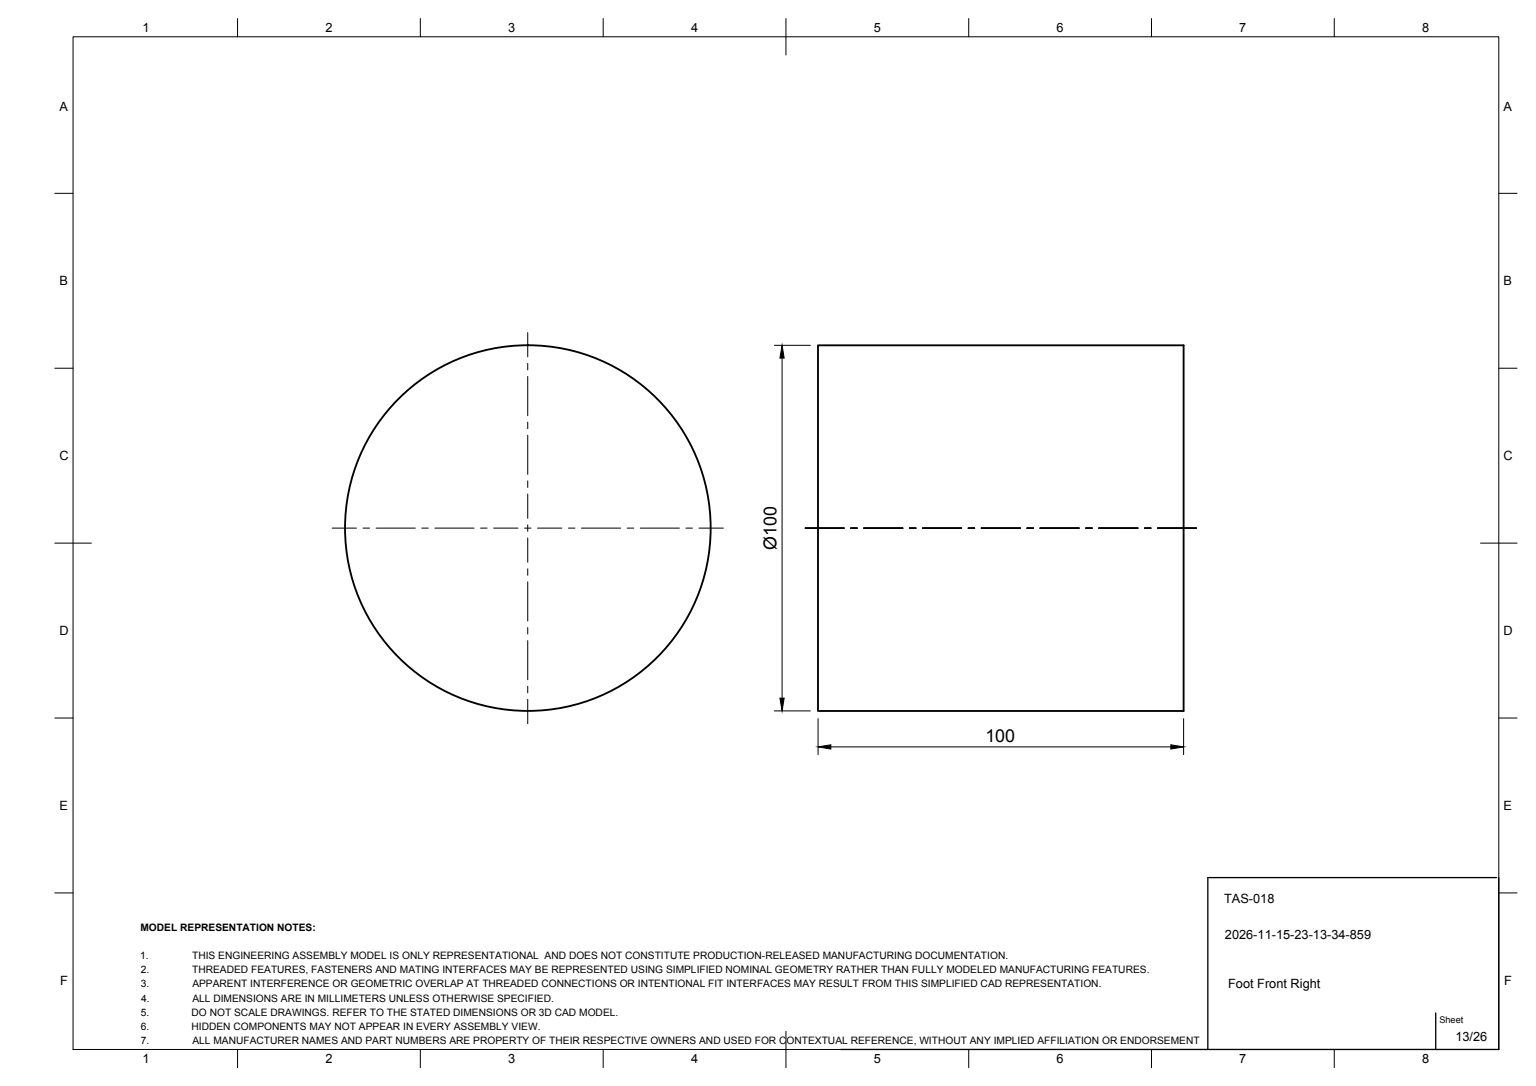
ISO-10303-21;
HEADER;
/* Generated by software containing ST-Developer
 * from STEP Tools, Inc. (www.steptools.com) 
 */

FILE_DESCRIPTION(
/* description */ (''),
/* implementation_level */ '2;1');

FILE_NAME(
/* name */ 'Foot Front Right.step',
/* time_stamp */ '2026-11-15T15:17:57-08:00',
/* author */ (''),
/* organization */ (''),
/* preprocessor_version */ 'ST-DEVELOPER v20.2',
/* originating_system */ 'Autodesk Translation Framework v15.17.0.0',
/* authorisation */ '');

FILE_SCHEMA (('AUTOMOTIVE_DESIGN { 1 0 10303 214 3 1 1 }'));
ENDSEC;

DATA;
#10=MECHANICAL_DESIGN_GEOMETRIC_PRESENTATION_REPRESENTATION('',(#188),#3723);
#13=CIRCLE('',#2395,1.96850393700787);
#14=CIRCLE('',#2396,1.96850393700787);
#24=CYLINDRICAL_SURFACE('',#2394,1.96850393700787);
#140=SHAPE_REPRESENTATION_RELATIONSHIP('SRR','None',#3821,#164);
#164=ADVANCED_BREP_SHAPE_REPRESENTATION('',(#212),#3710);
#188=STYLED_ITEM('',(#3945),#212);
#212=MANIFOLD_SOLID_BREP('Body1',#2036);
#288=FACE_OUTER_BOUND('',#414,.T.);
#289=FACE_OUTER_BOUND('',#415,.T.);
#290=FACE_OUTER_BOUND('',#416,.T.);
#414=EDGE_LOOP('',(#1557,#1558,#1559,#1560));
#415=EDGE_LOOP('',(#1561));
#416=EDGE_LOOP('',(#1562));
#598=LINE('',#3390,#820);
#820=VECTOR('',#2788,1.96850393700787);
#1003=VERTEX_POINT('',#3387);
#1004=VERTEX_POINT('',#3389);
#1200=EDGE_CURVE('',#1003,#1003,#13,.T.);
#1201=EDGE_CURVE('',#1003,#1004,#598,.T.);
#1202=EDGE_CURVE('',#1004,#1004,#14,.T.);
#1557=ORIENTED_EDGE('',*,*,#1200,.T.);
#1558=ORIENTED_EDGE('',*,*,#1201,.T.);
#1559=ORIENTED_EDGE('',*,*,#1202,.F.);
#1560=ORIENTED_EDGE('',*,*,#1201,.F.);
#1561=ORIENTED_EDGE('',*,*,#1202,.T.);
#1562=ORIENTED_EDGE('',*,*,#1200,.F.);
#1841=PLANE('',#2397);
#1842=PLANE('',#2398);
#1962=ADVANCED_FACE('',(#288),#24,.T.);
#1963=ADVANCED_FACE('',(#289),#1841,.T.);
#1964=ADVANCED_FACE('',(#290),#1842,.F.);
#2036=CLOSED_SHELL('',(#1962,#1963,#1964));
#2393=AXIS2_PLACEMENT_3D('',#3385,#2782,#2783);
#2394=AXIS2_PLACEMENT_3D('',#3386,#2784,#2785);
#2395=AXIS2_PLACEMENT_3D('',#3388,#2786,#2787);
#2396=AXIS2_PLACEMENT_3D('',#3391,#2789,#2790);
#2397=AXIS2_PLACEMENT_3D('',#3392,#2791,#2792);
#2398=AXIS2_PLACEMENT_3D('',#3393,#2793,#2794);
#2782=DIRECTION('axis',(0.,0.,1.));
#2783=DIRECTION('refdir',(1.,0.,0.));
#2784=DIRECTION('center_axis',(0.,1.,0.));
#2785=DIRECTION('ref_axis',(0.,0.,1.));
#2786=DIRECTION('center_axis',(0.,-1.,0.));
#2787=DIRECTION('ref_axis',(0.,0.,-1.));
#2788=DIRECTION('',(0.,-1.,0.));
#2789=DIRECTION('center_axis',(0.,-1.,0.));
#2790=DIRECTION('ref_axis',(0.,0.,-1.));
#2791=DIRECTION('center_axis',(0.,-1.,0.));
#2792=DIRECTION('ref_axis',(0.,0.,-1.));
#2793=DIRECTION('center_axis',(0.,-1.,0.));
#2794=DIRECTION('ref_axis',(0.,0.,-1.));
#3385=CARTESIAN_POINT('',(0.,0.,0.));
#3386=CARTESIAN_POINT('Origin',(33.6377952755905,-4.91732638859567E-15,
19.6377952755906));
#3387=CARTESIAN_POINT('',(33.6377952755905,3.93700787401574,17.6692913385827));
#3388=CARTESIAN_POINT('Origin',(33.6377952755905,3.93700787401574,19.6377952755906));
#3389=CARTESIAN_POINT('',(33.6377952755905,-4.91732638859567E-15,17.6692913385827));
#3390=CARTESIAN_POINT('',(33.6377952755905,-4.91732638859567E-15,17.6692913385827));
#3391=CARTESIAN_POINT('Origin',(33.6377952755905,-4.91732638859567E-15,
19.6377952755906));
#3392=CARTESIAN_POINT('Origin',(33.6377952755905,-4.91732638859567E-15,
19.6377952755906));
#3393=CARTESIAN_POINT('Origin',(33.6377952755905,3.93700787401574,19.6377952755906));
#3683=UNCERTAINTY_MEASURE_WITH_UNIT(LENGTH_MEASURE(0.000393700787401575),
#3725,'DISTANCE_ACCURACY_VALUE',
'Maximum model space distance between geometric entities at asserted c
onnectivities');
#3696=UNCERTAINTY_MEASURE_WITH_UNIT(LENGTH_MEASURE(0.000393700787401575),
#3725,'DISTANCE_ACCURACY_VALUE',
'Maximum model space distance between geometric entities at asserted c
onnectivities');
#3710=(
GEOMETRIC_REPRESENTATION_CONTEXT(3)
GLOBAL_UNCERTAINTY_ASSIGNED_CONTEXT((#3683))
GLOBAL_UNIT_ASSIGNED_CONTEXT((#3725,#3729,#3730))
REPRESENTATION_CONTEXT('','3D')
);
#3723=(
GEOMETRIC_REPRESENTATION_CONTEXT(3)
GLOBAL_UNCERTAINTY_ASSIGNED_CONTEXT((#3696))
GLOBAL_UNIT_ASSIGNED_CONTEXT((#3725,#3729,#3730))
REPRESENTATION_CONTEXT('','3D')
);
#3724=DIMENSIONAL_EXPONENTS(1.,0.,0.,0.,0.,0.,0.);
#3725=(
CONVERSION_BASED_UNIT('inch',#3728)
LENGTH_UNIT()
NAMED_UNIT(#3724)
);
#3726=(
LENGTH_UNIT()
NAMED_UNIT(*)
SI_UNIT(.MILLI.,.METRE.)
);
#3728=LENGTH_MEASURE_WITH_UNIT(LENGTH_MEASURE(25.4),#3726);
#3729=(
NAMED_UNIT(*)
PLANE_ANGLE_UNIT()
SI_UNIT($,.RADIAN.)
);
#3730=(
NAMED_UNIT(*)
SI_UNIT($,.STERADIAN.)
SOLID_ANGLE_UNIT()
);
#3744=SHAPE_DEFINITION_REPRESENTATION(#3771,#3821);
#3771=PRODUCT_DEFINITION_SHAPE('',$,#3848);
#3821=SHAPE_REPRESENTATION('',(#2393),#3710);
#3834=PRODUCT_DEFINITION_CONTEXT('part definition',#3914,'design');
#3848=PRODUCT_DEFINITION('2026-11-15-23-13-34-859','Foot Front Right',#3874,
#3834);
#3874=PRODUCT_DEFINITION_FORMATION('',$,#3929);
#3914=APPLICATION_CONTEXT(
'Core Data for Automotive Mechanical Design Process');
#3915=PRODUCT_CONTEXT('part definition',#3914,'mechanical');
#3929=PRODUCT('2026-11-15-23-13-34-859','Foot Front Right',$,(#3915));
#3945=PRESENTATION_STYLE_ASSIGNMENT((#3953));
#3953=SURFACE_STYLE_USAGE(.BOTH.,#3961);
#3961=SURFACE_SIDE_STYLE('',(#3969));
#3969=SURFACE_STYLE_FILL_AREA(#3977);
#3977=FILL_AREA_STYLE('Black',(#3985));
#3985=FILL_AREA_STYLE_COLOUR('Black',#3993);
#3993=COLOUR_RGB('Black',0.0784313725490196,0.0784313725490196,0.0784313725490196);
ENDSEC;
END-ISO-10303-21;
